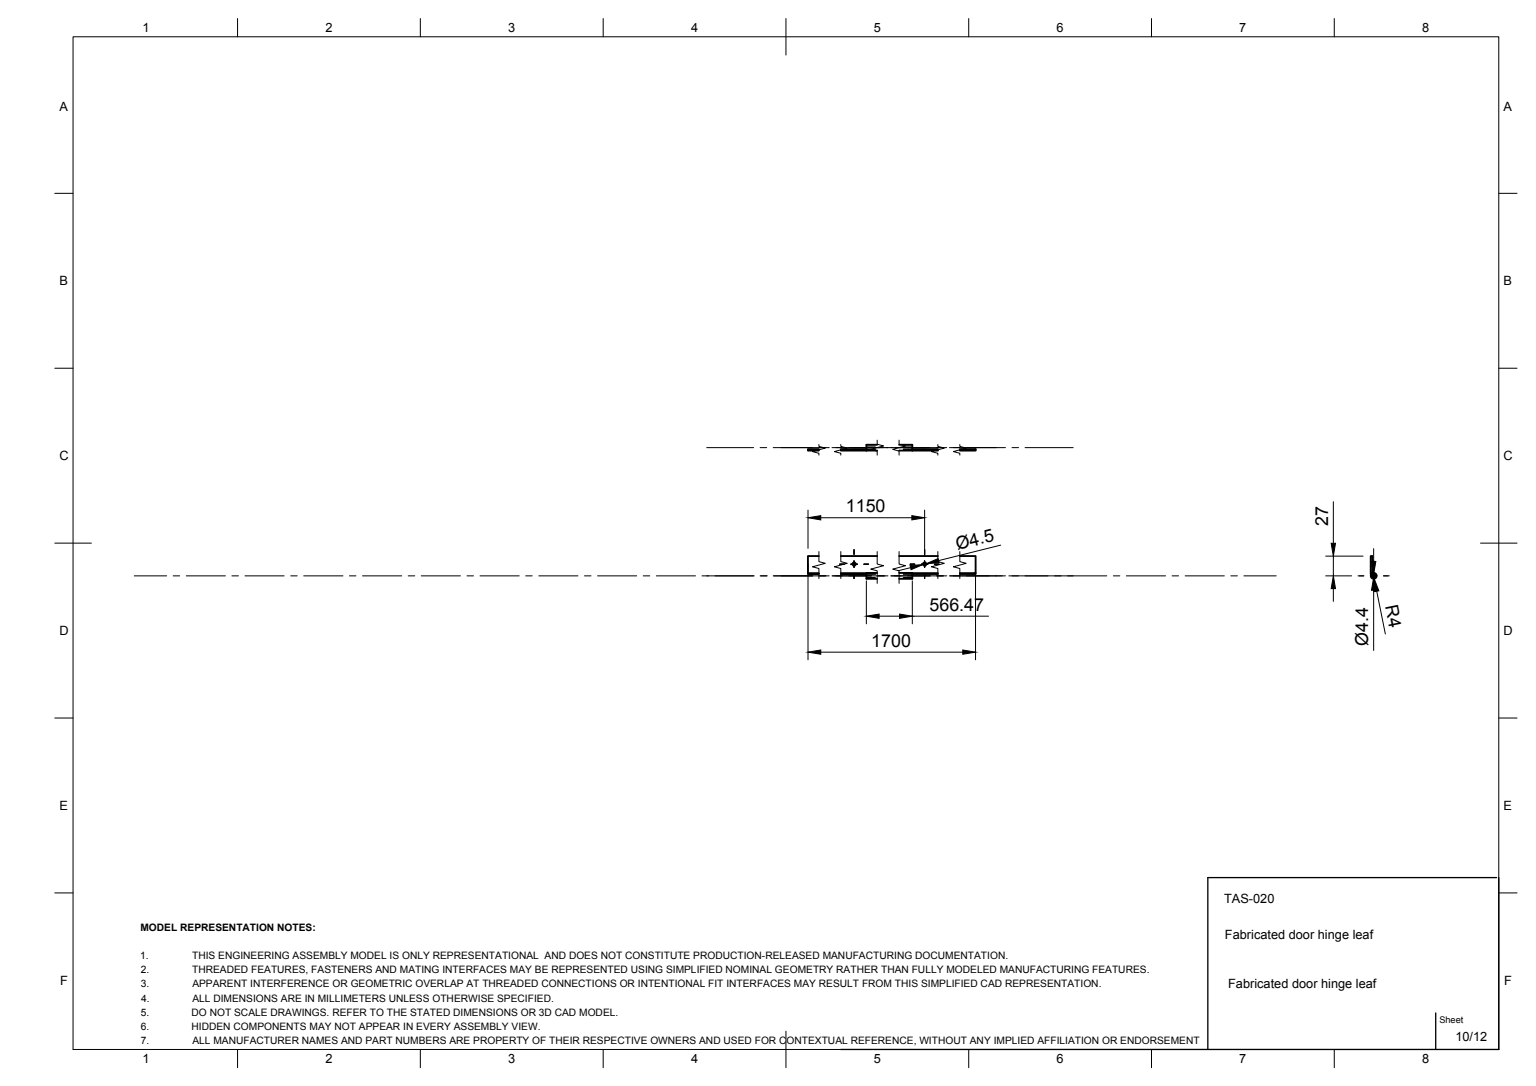
ISO-10303-21;
HEADER;
/* Generated by software containing ST-Developer
 * from STEP Tools, Inc. (www.steptools.com) 
 */

FILE_DESCRIPTION(
/* description */ (''),
/* implementation_level */ '2;1');

FILE_NAME(
/* name */ 'Fabricated door hinge leaf.step',
/* time_stamp */ '2026-11-15T17:46:57-08:00',
/* author */ (''),
/* organization */ (''),
/* preprocessor_version */ 'ST-DEVELOPER v20.2',
/* originating_system */ 'Autodesk Translation Framework v15.17.0.0',
/* authorisation */ '');

FILE_SCHEMA (('AUTOMOTIVE_DESIGN { 1 0 10303 214 3 1 1 }'));
ENDSEC;

DATA;
#10=MECHANICAL_DESIGN_GEOMETRIC_PRESENTATION_REPRESENTATION('',(#382),#12963);
#358=SHAPE_REPRESENTATION_RELATIONSHIP('SRR','None',#13042,#370);
#370=ADVANCED_BREP_SHAPE_REPRESENTATION('',(#394),#12958);
#382=STYLED_ITEM('',(#13111),#394);
#394=MANIFOLD_SOLID_BREP('Body1',#4816);
#429=FACE_BOUND('',#985,.T.);
#430=FACE_BOUND('',#986,.T.);
#431=FACE_BOUND('',#992,.T.);
#432=FACE_BOUND('',#996,.T.);
#433=FACE_BOUND('',#998,.T.);
#434=FACE_BOUND('',#999,.T.);
#538=PLANE('',#5141);
#539=PLANE('',#5145);
#540=PLANE('',#5146);
#541=PLANE('',#5150);
#542=PLANE('',#5151);
#543=PLANE('',#5152);
#544=PLANE('',#5159);
#545=PLANE('',#5160);
#546=PLANE('',#5161);
#547=PLANE('',#5162);
#694=FACE_OUTER_BOUND('',#980,.T.);
#695=FACE_OUTER_BOUND('',#981,.T.);
#696=FACE_OUTER_BOUND('',#982,.T.);
#697=FACE_OUTER_BOUND('',#983,.T.);
#698=FACE_OUTER_BOUND('',#984,.T.);
#699=FACE_OUTER_BOUND('',#987,.T.);
#700=FACE_OUTER_BOUND('',#988,.T.);
#701=FACE_OUTER_BOUND('',#989,.T.);
#702=FACE_OUTER_BOUND('',#990,.T.);
#703=FACE_OUTER_BOUND('',#991,.T.);
#704=FACE_OUTER_BOUND('',#993,.T.);
#705=FACE_OUTER_BOUND('',#994,.T.);
#706=FACE_OUTER_BOUND('',#995,.T.);
#707=FACE_OUTER_BOUND('',#997,.T.);
#708=FACE_OUTER_BOUND('',#1000,.T.);
#709=FACE_OUTER_BOUND('',#1001,.T.);
#980=EDGE_LOOP('',(#3712,#3713,#3714,#3715));
#981=EDGE_LOOP('',(#3716,#3717,#3718,#3719));
#982=EDGE_LOOP('',(#3720,#3721,#3722));
#983=EDGE_LOOP('',(#3723,#3724,#3725,#3726));
#984=EDGE_LOOP('',(#3727,#3728,#3729,#3730,#3731,#3732,#3733,#3734,#3735,
#3736,#3737,#3738));
#985=EDGE_LOOP('',(#3739));
#986=EDGE_LOOP('',(#3740));
#987=EDGE_LOOP('',(#3741,#3742,#3743,#3744,#3745,#3746,#3747,#3748,#3749,
#3750,#3751,#3752));
#988=EDGE_LOOP('',(#3753,#3754,#3755,#3756));
#989=EDGE_LOOP('',(#3757,#3758,#3759));
#990=EDGE_LOOP('',(#3760,#3761,#3762,#3763,#3764));
#991=EDGE_LOOP('',(#3765,#3766,#3767));
#992=EDGE_LOOP('',(#3768));
#993=EDGE_LOOP('',(#3769,#3770,#3771,#3772));
#994=EDGE_LOOP('',(#3773,#3774,#3775,#3776));
#995=EDGE_LOOP('',(#3777,#3778,#3779));
#996=EDGE_LOOP('',(#3780));
#997=EDGE_LOOP('',(#3781,#3782,#3783,#3784));
#998=EDGE_LOOP('',(#3785));
#999=EDGE_LOOP('',(#3786));
#1000=EDGE_LOOP('',(#3787,#3788,#3789,#3790));
#1001=EDGE_LOOP('',(#3791,#3792,#3793,#3794,#3795));
#1376=LINE('',#7152,#1778);
#1377=LINE('',#7158,#1779);
#1378=LINE('',#7163,#1780);
#1379=LINE('',#7166,#1781);
#1380=LINE('',#7169,#1782);
#1381=LINE('',#7172,#1783);
#1382=LINE('',#7175,#1784);
#1383=LINE('',#7177,#1785);
#1384=LINE('',#7179,#1786);
#1385=LINE('',#7181,#1787);
#1386=LINE('',#7183,#1788);
#1387=LINE('',#7185,#1789);
#1388=LINE('',#7187,#1790);
#1389=LINE('',#7189,#1791);
#1390=LINE('',#7191,#1792);
#1391=LINE('',#7192,#1793);
#1392=LINE('',#7195,#1794);
#1393=LINE('',#7197,#1795);
#1394=LINE('',#7199,#1796);
#1395=LINE('',#7201,#1797);
#1396=LINE('',#7202,#1798);
#1397=LINE('',#7204,#1799);
#1398=LINE('',#7206,#1800);
#1399=LINE('',#7207,#1801);
#1400=LINE('',#7214,#1802);
#1401=LINE('',#7215,#1803);
#1402=LINE('',#7222,#1804);
#1403=LINE('',#7229,#1805);
#1404=LINE('',#7230,#1806);
#1405=LINE('',#7232,#1807);
#1778=VECTOR('',#5957,0.225);
#1779=VECTOR('',#5964,0.225);
#1780=VECTOR('',#5969,1.);
#1781=VECTOR('',#5972,1.);
#1782=VECTOR('',#5975,1.);
#1783=VECTOR('',#5978,1.);
#1784=VECTOR('',#5981,1.);
#1785=VECTOR('',#5982,1.);
#1786=VECTOR('',#5983,1.);
#1787=VECTOR('',#5984,1.);
#1788=VECTOR('',#5985,1.);
#1789=VECTOR('',#5986,1.);
#1790=VECTOR('',#5987,1.);
#1791=VECTOR('',#5988,1.);
#1792=VECTOR('',#5989,1.);
#1793=VECTOR('',#5990,1.);
#1794=VECTOR('',#5993,1.);
#1795=VECTOR('',#5994,1.);
#1796=VECTOR('',#5995,1.);
#1797=VECTOR('',#5996,1.);
#1798=VECTOR('',#5997,1.);
#1799=VECTOR('',#5998,1.);
#1800=VECTOR('',#5999,1.);
#1801=VECTOR('',#6000,1.);
#1802=VECTOR('',#6011,1.);
#1803=VECTOR('',#6012,1.);
#1804=VECTOR('',#6021,0.22);
#1805=VECTOR('',#6032,1.);
#1806=VECTOR('',#6033,1.);
#1807=VECTOR('',#6036,1.);
#1980=CIRCLE('',#5136,0.225);
#1981=CIRCLE('',#5137,0.225);
#1982=CIRCLE('',#5139,0.225);
#1983=CIRCLE('',#5140,0.225);
#1984=CIRCLE('',#5142,0.42);
#1985=CIRCLE('',#5144,0.42);
#1986=CIRCLE('',#5148,0.42);
#1987=CIRCLE('',#5149,0.42);
#1988=CIRCLE('',#5153,0.4);
#1989=CIRCLE('',#5154,0.22);
#1990=CIRCLE('',#5156,0.22);
#1991=CIRCLE('',#5158,0.4);
#2212=VERTEX_POINT('',#7149);
#2213=VERTEX_POINT('',#7151);
#2214=VERTEX_POINT('',#7155);
#2215=VERTEX_POINT('',#7157);
#2216=VERTEX_POINT('',#7161);
#2217=VERTEX_POINT('',#7162);
#2218=VERTEX_POINT('',#7164);
#2219=VERTEX_POINT('',#7168);
#2220=VERTEX_POINT('',#7170);
#2221=VERTEX_POINT('',#7174);
#2222=VERTEX_POINT('',#7176);
#2223=VERTEX_POINT('',#7178);
#2224=VERTEX_POINT('',#7180);
#2225=VERTEX_POINT('',#7182);
#2226=VERTEX_POINT('',#7184);
#2227=VERTEX_POINT('',#7186);
#2228=VERTEX_POINT('',#7188);
#2229=VERTEX_POINT('',#7190);
#2230=VERTEX_POINT('',#7194);
#2231=VERTEX_POINT('',#7196);
#2232=VERTEX_POINT('',#7198);
#2233=VERTEX_POINT('',#7200);
#2234=VERTEX_POINT('',#7203);
#2235=VERTEX_POINT('',#7205);
#2236=VERTEX_POINT('',#7213);
#2237=VERTEX_POINT('',#7218);
#2238=VERTEX_POINT('',#7221);
#2239=VERTEX_POINT('',#7228);
#2752=EDGE_CURVE('',#2212,#2212,#1980,.T.);
#2753=EDGE_CURVE('',#2212,#2213,#1376,.T.);
#2754=EDGE_CURVE('',#2213,#2213,#1981,.T.);
#2755=EDGE_CURVE('',#2214,#2214,#1982,.T.);
#2756=EDGE_CURVE('',#2214,#2215,#1377,.T.);
#2757=EDGE_CURVE('',#2215,#2215,#1983,.T.);
#2758=EDGE_CURVE('',#2216,#2217,#1378,.T.);
#2759=EDGE_CURVE('',#2216,#2218,#1984,.T.);
#2760=EDGE_CURVE('',#2217,#2218,#1379,.T.);
#2761=EDGE_CURVE('',#2219,#2216,#1380,.T.);
#2762=EDGE_CURVE('',#2220,#2219,#1985,.T.);
#2763=EDGE_CURVE('',#2218,#2220,#1381,.T.);
#2764=EDGE_CURVE('',#2221,#2217,#1382,.T.);
#2765=EDGE_CURVE('',#2221,#2222,#1383,.T.);
#2766=EDGE_CURVE('',#2222,#2223,#1384,.T.);
#2767=EDGE_CURVE('',#2223,#2224,#1385,.T.);
#2768=EDGE_CURVE('',#2225,#2224,#1386,.T.);
#2769=EDGE_CURVE('',#2225,#2226,#1387,.T.);
#2770=EDGE_CURVE('',#2226,#2227,#1388,.T.);
#2771=EDGE_CURVE('',#2227,#2228,#1389,.T.);
#2772=EDGE_CURVE('',#2228,#2229,#1390,.T.);
#2773=EDGE_CURVE('',#2219,#2229,#1391,.T.);
#2774=EDGE_CURVE('',#2230,#2220,#1392,.T.);
#2775=EDGE_CURVE('',#2231,#2230,#1393,.T.);
#2776=EDGE_CURVE('',#2231,#2232,#1394,.T.);
#2777=EDGE_CURVE('',#2232,#2233,#1395,.T.);
#2778=EDGE_CURVE('',#2233,#2225,#1396,.T.);
#2779=EDGE_CURVE('',#2224,#2234,#1397,.T.);
#2780=EDGE_CURVE('',#2234,#2235,#1398,.T.);
#2781=EDGE_CURVE('',#2235,#2221,#1399,.T.);
#2782=EDGE_CURVE('',#2226,#2233,#1986,.T.);
#2783=EDGE_CURVE('',#2227,#2232,#1987,.T.);
#2784=EDGE_CURVE('',#2236,#2231,#1400,.T.);
#2785=EDGE_CURVE('',#2228,#2236,#1401,.T.);
#2786=EDGE_CURVE('',#2235,#2222,#1988,.T.);
#2787=EDGE_CURVE('',#2237,#2237,#1989,.T.);
#2788=EDGE_CURVE('',#2237,#2238,#1402,.T.);
#2789=EDGE_CURVE('',#2238,#2238,#1990,.T.);
#2790=EDGE_CURVE('',#2234,#2223,#1991,.T.);
#2791=EDGE_CURVE('',#2239,#2230,#1403,.T.);
#2792=EDGE_CURVE('',#2236,#2239,#1404,.T.);
#2793=EDGE_CURVE('',#2229,#2239,#1405,.T.);
#3712=ORIENTED_EDGE('',*,*,#2752,.F.);
#3713=ORIENTED_EDGE('',*,*,#2753,.T.);
#3714=ORIENTED_EDGE('',*,*,#2754,.F.);
#3715=ORIENTED_EDGE('',*,*,#2753,.F.);
#3716=ORIENTED_EDGE('',*,*,#2755,.F.);
#3717=ORIENTED_EDGE('',*,*,#2756,.T.);
#3718=ORIENTED_EDGE('',*,*,#2757,.F.);
#3719=ORIENTED_EDGE('',*,*,#2756,.F.);
#3720=ORIENTED_EDGE('',*,*,#2758,.F.);
#3721=ORIENTED_EDGE('',*,*,#2759,.T.);
#3722=ORIENTED_EDGE('',*,*,#2760,.F.);
#3723=ORIENTED_EDGE('',*,*,#2761,.F.);
#3724=ORIENTED_EDGE('',*,*,#2762,.F.);
#3725=ORIENTED_EDGE('',*,*,#2763,.F.);
#3726=ORIENTED_EDGE('',*,*,#2759,.F.);
#3727=ORIENTED_EDGE('',*,*,#2761,.T.);
#3728=ORIENTED_EDGE('',*,*,#2758,.T.);
#3729=ORIENTED_EDGE('',*,*,#2764,.F.);
#3730=ORIENTED_EDGE('',*,*,#2765,.T.);
#3731=ORIENTED_EDGE('',*,*,#2766,.T.);
#3732=ORIENTED_EDGE('',*,*,#2767,.T.);
#3733=ORIENTED_EDGE('',*,*,#2768,.F.);
#3734=ORIENTED_EDGE('',*,*,#2769,.T.);
#3735=ORIENTED_EDGE('',*,*,#2770,.T.);
#3736=ORIENTED_EDGE('',*,*,#2771,.T.);
#3737=ORIENTED_EDGE('',*,*,#2772,.T.);
#3738=ORIENTED_EDGE('',*,*,#2773,.F.);
#3739=ORIENTED_EDGE('',*,*,#2754,.T.);
#3740=ORIENTED_EDGE('',*,*,#2757,.T.);
#3741=ORIENTED_EDGE('',*,*,#2760,.T.);
#3742=ORIENTED_EDGE('',*,*,#2763,.T.);
#3743=ORIENTED_EDGE('',*,*,#2774,.F.);
#3744=ORIENTED_EDGE('',*,*,#2775,.F.);
#3745=ORIENTED_EDGE('',*,*,#2776,.T.);
#3746=ORIENTED_EDGE('',*,*,#2777,.T.);
#3747=ORIENTED_EDGE('',*,*,#2778,.T.);
#3748=ORIENTED_EDGE('',*,*,#2768,.T.);
#3749=ORIENTED_EDGE('',*,*,#2779,.T.);
#3750=ORIENTED_EDGE('',*,*,#2780,.T.);
#3751=ORIENTED_EDGE('',*,*,#2781,.T.);
#3752=ORIENTED_EDGE('',*,*,#2764,.T.);
#3753=ORIENTED_EDGE('',*,*,#2770,.F.);
#3754=ORIENTED_EDGE('',*,*,#2782,.T.);
#3755=ORIENTED_EDGE('',*,*,#2777,.F.);
#3756=ORIENTED_EDGE('',*,*,#2783,.F.);
#3757=ORIENTED_EDGE('',*,*,#2769,.F.);
#3758=ORIENTED_EDGE('',*,*,#2778,.F.);
#3759=ORIENTED_EDGE('',*,*,#2782,.F.);
#3760=ORIENTED_EDGE('',*,*,#2783,.T.);
#3761=ORIENTED_EDGE('',*,*,#2776,.F.);
#3762=ORIENTED_EDGE('',*,*,#2784,.F.);
#3763=ORIENTED_EDGE('',*,*,#2785,.F.);
#3764=ORIENTED_EDGE('',*,*,#2771,.F.);
#3765=ORIENTED_EDGE('',*,*,#2765,.F.);
#3766=ORIENTED_EDGE('',*,*,#2781,.F.);
#3767=ORIENTED_EDGE('',*,*,#2786,.T.);
#3768=ORIENTED_EDGE('',*,*,#2787,.T.);
#3769=ORIENTED_EDGE('',*,*,#2787,.F.);
#3770=ORIENTED_EDGE('',*,*,#2788,.T.);
#3771=ORIENTED_EDGE('',*,*,#2789,.T.);
#3772=ORIENTED_EDGE('',*,*,#2788,.F.);
#3773=ORIENTED_EDGE('',*,*,#2766,.F.);
#3774=ORIENTED_EDGE('',*,*,#2786,.F.);
#3775=ORIENTED_EDGE('',*,*,#2780,.F.);
#3776=ORIENTED_EDGE('',*,*,#2790,.T.);
#3777=ORIENTED_EDGE('',*,*,#2767,.F.);
#3778=ORIENTED_EDGE('',*,*,#2790,.F.);
#3779=ORIENTED_EDGE('',*,*,#2779,.F.);
#3780=ORIENTED_EDGE('',*,*,#2789,.F.);
#3781=ORIENTED_EDGE('',*,*,#2784,.T.);
#3782=ORIENTED_EDGE('',*,*,#2775,.T.);
#3783=ORIENTED_EDGE('',*,*,#2791,.F.);
#3784=ORIENTED_EDGE('',*,*,#2792,.F.);
#3785=ORIENTED_EDGE('',*,*,#2752,.T.);
#3786=ORIENTED_EDGE('',*,*,#2755,.T.);
#3787=ORIENTED_EDGE('',*,*,#2785,.T.);
#3788=ORIENTED_EDGE('',*,*,#2792,.T.);
#3789=ORIENTED_EDGE('',*,*,#2793,.F.);
#3790=ORIENTED_EDGE('',*,*,#2772,.F.);
#3791=ORIENTED_EDGE('',*,*,#2762,.T.);
#3792=ORIENTED_EDGE('',*,*,#2773,.T.);
#3793=ORIENTED_EDGE('',*,*,#2793,.T.);
#3794=ORIENTED_EDGE('',*,*,#2791,.T.);
#3795=ORIENTED_EDGE('',*,*,#2774,.T.);
#4457=CYLINDRICAL_SURFACE('',#5135,0.225);
#4458=CYLINDRICAL_SURFACE('',#5138,0.225);
#4459=CYLINDRICAL_SURFACE('',#5143,0.42);
#4460=CYLINDRICAL_SURFACE('',#5147,0.42);
#4461=CYLINDRICAL_SURFACE('',#5155,0.22);
#4462=CYLINDRICAL_SURFACE('',#5157,0.4);
#4675=ADVANCED_FACE('',(#694),#4457,.F.);
#4676=ADVANCED_FACE('',(#695),#4458,.F.);
#4677=ADVANCED_FACE('',(#696),#538,.T.);
#4678=ADVANCED_FACE('',(#697),#4459,.F.);
#4679=ADVANCED_FACE('',(#698,#429,#430),#539,.T.);
#4680=ADVANCED_FACE('',(#699),#540,.T.);
#4681=ADVANCED_FACE('',(#700),#4460,.F.);
#4682=ADVANCED_FACE('',(#701),#541,.F.);
#4683=ADVANCED_FACE('',(#702),#542,.F.);
#4684=ADVANCED_FACE('',(#703,#431),#543,.T.);
#4685=ADVANCED_FACE('',(#704),#4461,.F.);
#4686=ADVANCED_FACE('',(#705),#4462,.T.);
#4687=ADVANCED_FACE('',(#706,#432),#544,.F.);
#4688=ADVANCED_FACE('',(#707,#433,#434),#545,.T.);
#4689=ADVANCED_FACE('',(#708),#546,.T.);
#4690=ADVANCED_FACE('',(#709),#547,.T.);
#4816=CLOSED_SHELL('',(#4675,#4676,#4677,#4678,#4679,#4680,#4681,#4682,
#4683,#4684,#4685,#4686,#4687,#4688,#4689,#4690));
#5134=AXIS2_PLACEMENT_3D('',#7147,#5951,#5952);
#5135=AXIS2_PLACEMENT_3D('',#7148,#5953,#5954);
#5136=AXIS2_PLACEMENT_3D('',#7150,#5955,#5956);
#5137=AXIS2_PLACEMENT_3D('',#7153,#5958,#5959);
#5138=AXIS2_PLACEMENT_3D('',#7154,#5960,#5961);
#5139=AXIS2_PLACEMENT_3D('',#7156,#5962,#5963);
#5140=AXIS2_PLACEMENT_3D('',#7159,#5965,#5966);
#5141=AXIS2_PLACEMENT_3D('',#7160,#5967,#5968);
#5142=AXIS2_PLACEMENT_3D('',#7165,#5970,#5971);
#5143=AXIS2_PLACEMENT_3D('',#7167,#5973,#5974);
#5144=AXIS2_PLACEMENT_3D('',#7171,#5976,#5977);
#5145=AXIS2_PLACEMENT_3D('',#7173,#5979,#5980);
#5146=AXIS2_PLACEMENT_3D('',#7193,#5991,#5992);
#5147=AXIS2_PLACEMENT_3D('',#7208,#6001,#6002);
#5148=AXIS2_PLACEMENT_3D('',#7209,#6003,#6004);
#5149=AXIS2_PLACEMENT_3D('',#7210,#6005,#6006);
#5150=AXIS2_PLACEMENT_3D('',#7211,#6007,#6008);
#5151=AXIS2_PLACEMENT_3D('',#7212,#6009,#6010);
#5152=AXIS2_PLACEMENT_3D('',#7216,#6013,#6014);
#5153=AXIS2_PLACEMENT_3D('',#7217,#6015,#6016);
#5154=AXIS2_PLACEMENT_3D('',#7219,#6017,#6018);
#5155=AXIS2_PLACEMENT_3D('',#7220,#6019,#6020);
#5156=AXIS2_PLACEMENT_3D('',#7223,#6022,#6023);
#5157=AXIS2_PLACEMENT_3D('',#7224,#6024,#6025);
#5158=AXIS2_PLACEMENT_3D('',#7225,#6026,#6027);
#5159=AXIS2_PLACEMENT_3D('',#7226,#6028,#6029);
#5160=AXIS2_PLACEMENT_3D('',#7227,#6030,#6031);
#5161=AXIS2_PLACEMENT_3D('',#7231,#6034,#6035);
#5162=AXIS2_PLACEMENT_3D('',#7233,#6037,#6038);
#5951=DIRECTION('axis',(0.,0.,1.));
#5952=DIRECTION('refdir',(1.,0.,0.));
#5953=DIRECTION('center_axis',(0.,-1.,0.));
#5954=DIRECTION('ref_axis',(1.,0.,0.));
#5955=DIRECTION('center_axis',(0.,-1.,0.));
#5956=DIRECTION('ref_axis',(1.,0.,0.));
#5957=DIRECTION('',(0.,-1.,0.));
#5958=DIRECTION('center_axis',(0.,1.,0.));
#5959=DIRECTION('ref_axis',(1.,0.,0.));
#5960=DIRECTION('center_axis',(0.,-1.,0.));
#5961=DIRECTION('ref_axis',(1.,0.,0.));
#5962=DIRECTION('center_axis',(0.,-1.,0.));
#5963=DIRECTION('ref_axis',(1.,0.,0.));
#5964=DIRECTION('',(0.,-1.,0.));
#5965=DIRECTION('center_axis',(0.,1.,0.));
#5966=DIRECTION('ref_axis',(1.,0.,0.));
#5967=DIRECTION('center_axis',(0.,0.,1.));
#5968=DIRECTION('ref_axis',(1.,0.,0.));
#5969=DIRECTION('',(-1.,0.,0.));
#5970=DIRECTION('center_axis',(0.,0.,1.));
#5971=DIRECTION('ref_axis',(1.,0.,0.));
#5972=DIRECTION('',(0.,1.,0.));
#5973=DIRECTION('center_axis',(0.,0.,1.));
#5974=DIRECTION('ref_axis',(1.,0.,0.));
#5975=DIRECTION('',(0.,0.,-1.));
#5976=DIRECTION('center_axis',(0.,0.,-1.));
#5977=DIRECTION('ref_axis',(1.,0.,0.));
#5978=DIRECTION('',(0.,0.,1.));
#5979=DIRECTION('center_axis',(0.,-1.,0.));
#5980=DIRECTION('ref_axis',(1.,0.,0.));
#5981=DIRECTION('',(0.,0.,1.));
#5982=DIRECTION('',(1.,0.,0.));
#5983=DIRECTION('',(0.,0.,-1.));
#5984=DIRECTION('',(-1.,0.,0.));
#5985=DIRECTION('',(0.,0.,1.));
#5986=DIRECTION('',(1.,0.,0.));
#5987=DIRECTION('',(0.,0.,-1.));
#5988=DIRECTION('',(1.,0.,0.));
#5989=DIRECTION('',(0.,0.,1.));
#5990=DIRECTION('',(1.,0.,0.));
#5991=DIRECTION('center_axis',(-1.,0.,0.));
#5992=DIRECTION('ref_axis',(0.,-1.,0.));
#5993=DIRECTION('',(0.,-1.,0.));
#5994=DIRECTION('',(0.,0.,1.));
#5995=DIRECTION('',(0.,-1.,0.));
#5996=DIRECTION('',(0.,0.,1.));
#5997=DIRECTION('',(0.,-1.,0.));
#5998=DIRECTION('',(0.,1.,0.));
#5999=DIRECTION('',(0.,0.,1.));
#6000=DIRECTION('',(0.,-1.,0.));
#6001=DIRECTION('center_axis',(0.,0.,1.));
#6002=DIRECTION('ref_axis',(1.,0.,0.));
#6003=DIRECTION('center_axis',(0.,0.,1.));
#6004=DIRECTION('ref_axis',(1.,0.,0.));
#6005=DIRECTION('center_axis',(0.,0.,1.));
#6006=DIRECTION('ref_axis',(1.,0.,0.));
#6007=DIRECTION('center_axis',(0.,0.,1.));
#6008=DIRECTION('ref_axis',(1.,0.,0.));
#6009=DIRECTION('center_axis',(0.,0.,1.));
#6010=DIRECTION('ref_axis',(1.,0.,0.));
#6011=DIRECTION('',(-1.,0.,0.));
#6012=DIRECTION('',(0.,1.,0.));
#6013=DIRECTION('center_axis',(0.,0.,1.));
#6014=DIRECTION('ref_axis',(1.,0.,0.));
#6015=DIRECTION('center_axis',(0.,0.,1.));
#6016=DIRECTION('ref_axis',(1.,0.,0.));
#6017=DIRECTION('center_axis',(0.,0.,-1.));
#6018=DIRECTION('ref_axis',(1.,0.,0.));
#6019=DIRECTION('center_axis',(0.,0.,1.));
#6020=DIRECTION('ref_axis',(1.,0.,0.));
#6021=DIRECTION('',(0.,0.,-1.));
#6022=DIRECTION('center_axis',(0.,0.,-1.));
#6023=DIRECTION('ref_axis',(1.,0.,0.));
#6024=DIRECTION('center_axis',(0.,0.,1.));
#6025=DIRECTION('ref_axis',(-0.758601839724033,-0.651554486414845,0.));
#6026=DIRECTION('center_axis',(0.,0.,1.));
#6027=DIRECTION('ref_axis',(1.,0.,0.));
#6028=DIRECTION('center_axis',(0.,0.,1.));
#6029=DIRECTION('ref_axis',(1.,0.,0.));
#6030=DIRECTION('center_axis',(0.,1.,0.));
#6031=DIRECTION('ref_axis',(-1.,0.,0.));
#6032=DIRECTION('',(-1.,0.,0.));
#6033=DIRECTION('',(0.,0.,1.));
#6034=DIRECTION('center_axis',(1.,0.,0.));
#6035=DIRECTION('ref_axis',(0.,1.,0.));
#6036=DIRECTION('',(0.,1.,0.));
#6037=DIRECTION('center_axis',(0.,0.,1.));
#6038=DIRECTION('ref_axis',(1.,0.,0.));
#7147=CARTESIAN_POINT('',(0.,0.,0.));
#7148=CARTESIAN_POINT('Origin',(1.6,0.4,55.));
#7149=CARTESIAN_POINT('',(1.375,0.4,55.));
#7150=CARTESIAN_POINT('Origin',(1.6,0.4,55.));
#7151=CARTESIAN_POINT('',(1.375,0.2,55.));
#7152=CARTESIAN_POINT('',(1.375,0.4,55.));
#7153=CARTESIAN_POINT('Origin',(1.6,0.2,55.));
#7154=CARTESIAN_POINT('Origin',(1.6,0.4,115.));
#7155=CARTESIAN_POINT('',(1.375,0.4,115.));
#7156=CARTESIAN_POINT('Origin',(1.6,0.4,115.));
#7157=CARTESIAN_POINT('',(1.375,0.2,115.));
#7158=CARTESIAN_POINT('',(1.375,0.4,115.));
#7159=CARTESIAN_POINT('Origin',(1.6,0.2,115.));
#7160=CARTESIAN_POINT('Origin',(0.,0.,113.323333333333));
#7161=CARTESIAN_POINT('',(0.369323706252388,0.2,113.323333333333));
#7162=CARTESIAN_POINT('',(0.25,0.2,113.323333333333));
#7163=CARTESIAN_POINT('',(0.125,0.2,113.323333333333));
#7164=CARTESIAN_POINT('',(0.25,0.337490740613724,113.323333333333));
#7165=CARTESIAN_POINT('Origin',(0.,0.,113.323333333333));
#7166=CARTESIAN_POINT('',(0.25,0.2,113.323333333333));
#7167=CARTESIAN_POINT('Origin',(0.,0.,113.323333333333));
#7168=CARTESIAN_POINT('',(0.369323706252388,0.2,170.));
#7169=CARTESIAN_POINT('',(0.369323706252388,0.2,113.323333333333));
#7170=CARTESIAN_POINT('',(0.25,0.337490740613724,170.));
#7171=CARTESIAN_POINT('Origin',(0.,0.,170.));
#7172=CARTESIAN_POINT('',(0.25,0.337490740613724,113.323333333333));
#7173=CARTESIAN_POINT('Origin',(0.25,0.2,0.));
#7174=CARTESIAN_POINT('',(0.25,0.2,113.313333333333));
#7175=CARTESIAN_POINT('',(0.25,0.2,0.));
#7176=CARTESIAN_POINT('',(0.346410161513776,0.2,113.313333333333));
#7177=CARTESIAN_POINT('',(0.125,0.2,113.313333333333));
#7178=CARTESIAN_POINT('',(0.346410161513776,0.2,56.6866666666667));
#7179=CARTESIAN_POINT('',(0.346410161513776,0.2,56.6866666666667));
#7180=CARTESIAN_POINT('',(0.25,0.2,56.6866666666667));
#7181=CARTESIAN_POINT('',(0.125,0.2,56.6866666666667));
#7182=CARTESIAN_POINT('',(0.25,0.2,56.6766666666667));
#7183=CARTESIAN_POINT('',(0.25,0.2,0.));
#7184=CARTESIAN_POINT('',(0.369323706252388,0.2,56.6766666666667));
#7185=CARTESIAN_POINT('',(0.125,0.2,56.6766666666667));
#7186=CARTESIAN_POINT('',(0.369323706252388,0.2,0.));
#7187=CARTESIAN_POINT('',(0.369323706252388,0.2,0.));
#7188=CARTESIAN_POINT('',(2.7,0.2,0.));
#7189=CARTESIAN_POINT('',(0.25,0.2,0.));
#7190=CARTESIAN_POINT('',(2.7,0.2,170.));
#7191=CARTESIAN_POINT('',(2.7,0.2,0.));
#7192=CARTESIAN_POINT('',(0.25,0.2,170.));
#7193=CARTESIAN_POINT('Origin',(0.25,0.4,0.));
#7194=CARTESIAN_POINT('',(0.25,0.4,170.));
#7195=CARTESIAN_POINT('',(0.25,0.4,170.));
#7196=CARTESIAN_POINT('',(0.25,0.4,0.));
#7197=CARTESIAN_POINT('',(0.25,0.4,0.));
#7198=CARTESIAN_POINT('',(0.25,0.337490740613724,0.));
#7199=CARTESIAN_POINT('',(0.25,0.4,0.));
#7200=CARTESIAN_POINT('',(0.25,0.337490740613724,56.6766666666667));
#7201=CARTESIAN_POINT('',(0.25,0.337490740613724,0.));
#7202=CARTESIAN_POINT('',(0.25,0.2,56.6766666666667));
#7203=CARTESIAN_POINT('',(0.25,0.31224989991992,56.6866666666667));
#7204=CARTESIAN_POINT('',(0.25,0.2,56.6866666666667));
#7205=CARTESIAN_POINT('',(0.25,0.31224989991992,113.313333333333));
#7206=CARTESIAN_POINT('',(0.25,0.31224989991992,56.6866666666667));
#7207=CARTESIAN_POINT('',(0.25,0.2,113.313333333333));
#7208=CARTESIAN_POINT('Origin',(0.,0.,0.));
#7209=CARTESIAN_POINT('Origin',(0.,0.,56.6766666666667));
#7210=CARTESIAN_POINT('Origin',(0.,0.,0.));
#7211=CARTESIAN_POINT('Origin',(0.,0.,56.6766666666667));
#7212=CARTESIAN_POINT('Origin',(1.475,0.3,0.));
#7213=CARTESIAN_POINT('',(2.7,0.4,0.));
#7214=CARTESIAN_POINT('',(2.7,0.4,0.));
#7215=CARTESIAN_POINT('',(2.7,0.2,0.));
#7216=CARTESIAN_POINT('Origin',(0.,0.,113.313333333333));
#7217=CARTESIAN_POINT('Origin',(0.,0.,113.313333333333));
#7218=CARTESIAN_POINT('',(-0.22,-2.69422295812418E-17,113.313333333333));
#7219=CARTESIAN_POINT('Origin',(0.,0.,113.313333333333));
#7220=CARTESIAN_POINT('Origin',(0.,0.,56.6866666666667));
#7221=CARTESIAN_POINT('',(-0.22,-2.69422295812418E-17,56.6866666666667));
#7222=CARTESIAN_POINT('',(-0.22,-2.69422295812418E-17,56.6866666666667));
#7223=CARTESIAN_POINT('Origin',(0.,0.,56.6866666666667));
#7224=CARTESIAN_POINT('Origin',(0.,0.,56.6866666666667));
#7225=CARTESIAN_POINT('Origin',(0.,0.,56.6866666666667));
#7226=CARTESIAN_POINT('Origin',(0.,0.,56.6866666666667));
#7227=CARTESIAN_POINT('Origin',(2.7,0.4,0.));
#7228=CARTESIAN_POINT('',(2.7,0.4,170.));
#7229=CARTESIAN_POINT('',(2.7,0.4,170.));
#7230=CARTESIAN_POINT('',(2.7,0.4,0.));
#7231=CARTESIAN_POINT('Origin',(2.7,0.2,0.));
#7232=CARTESIAN_POINT('',(2.7,0.2,170.));
#7233=CARTESIAN_POINT('Origin',(1.475,0.3,170.));
#12944=UNCERTAINTY_MEASURE_WITH_UNIT(LENGTH_MEASURE(0.001),#12964,
'DISTANCE_ACCURACY_VALUE',
'Maximum model space distance between geometric entities at asserted c
onnectivities');
#12949=UNCERTAINTY_MEASURE_WITH_UNIT(LENGTH_MEASURE(0.001),#12964,
'DISTANCE_ACCURACY_VALUE',
'Maximum model space distance between geometric entities at asserted c
onnectivities');
#12958=(
GEOMETRIC_REPRESENTATION_CONTEXT(3)
GLOBAL_UNCERTAINTY_ASSIGNED_CONTEXT((#12944))
GLOBAL_UNIT_ASSIGNED_CONTEXT((#12964,#12966,#12967))
REPRESENTATION_CONTEXT('','3D')
);
#12963=(
GEOMETRIC_REPRESENTATION_CONTEXT(3)
GLOBAL_UNCERTAINTY_ASSIGNED_CONTEXT((#12949))
GLOBAL_UNIT_ASSIGNED_CONTEXT((#12964,#12966,#12967))
REPRESENTATION_CONTEXT('','3D')
);
#12964=(
LENGTH_UNIT()
NAMED_UNIT(*)
SI_UNIT(.CENTI.,.METRE.)
);
#12966=(
NAMED_UNIT(*)
PLANE_ANGLE_UNIT()
SI_UNIT($,.RADIAN.)
);
#12967=(
NAMED_UNIT(*)
SI_UNIT($,.STERADIAN.)
SOLID_ANGLE_UNIT()
);
#12976=SHAPE_DEFINITION_REPRESENTATION(#12989,#13042);
#12989=PRODUCT_DEFINITION_SHAPE('',$,#13056);
#13042=SHAPE_REPRESENTATION('',(#5134),#12958);
#13047=PRODUCT_DEFINITION_CONTEXT('part definition',#13088,'design');
#13056=PRODUCT_DEFINITION('Fabricated door hinge leaf',
'Fabricated door hinge leaf',#13069,#13047);
#13069=PRODUCT_DEFINITION_FORMATION('',$,#13098);
#13088=APPLICATION_CONTEXT(
'Core Data for Automotive Mechanical Design Process');
#13089=PRODUCT_CONTEXT('part definition',#13088,'mechanical');
#13098=PRODUCT('Fabricated door hinge leaf',
'Fabricated door hinge leaf',$,(#13089));
#13111=PRESENTATION_STYLE_ASSIGNMENT((#13124));
#13124=SURFACE_STYLE_USAGE(.BOTH.,#13137);
#13137=SURFACE_SIDE_STYLE('',(#13150));
#13150=SURFACE_STYLE_FILL_AREA(#13163);
#13163=FILL_AREA_STYLE('Fabricated door hinge leaf finish',(#13176));
#13176=FILL_AREA_STYLE_COLOUR('Fabricated door hinge leaf finish',#13189);
#13189=COLOUR_RGB('Fabricated door hinge leaf finish',0.607843137254902,
0.647058823529412,0.701960784313725);
ENDSEC;
END-ISO-10303-21;
